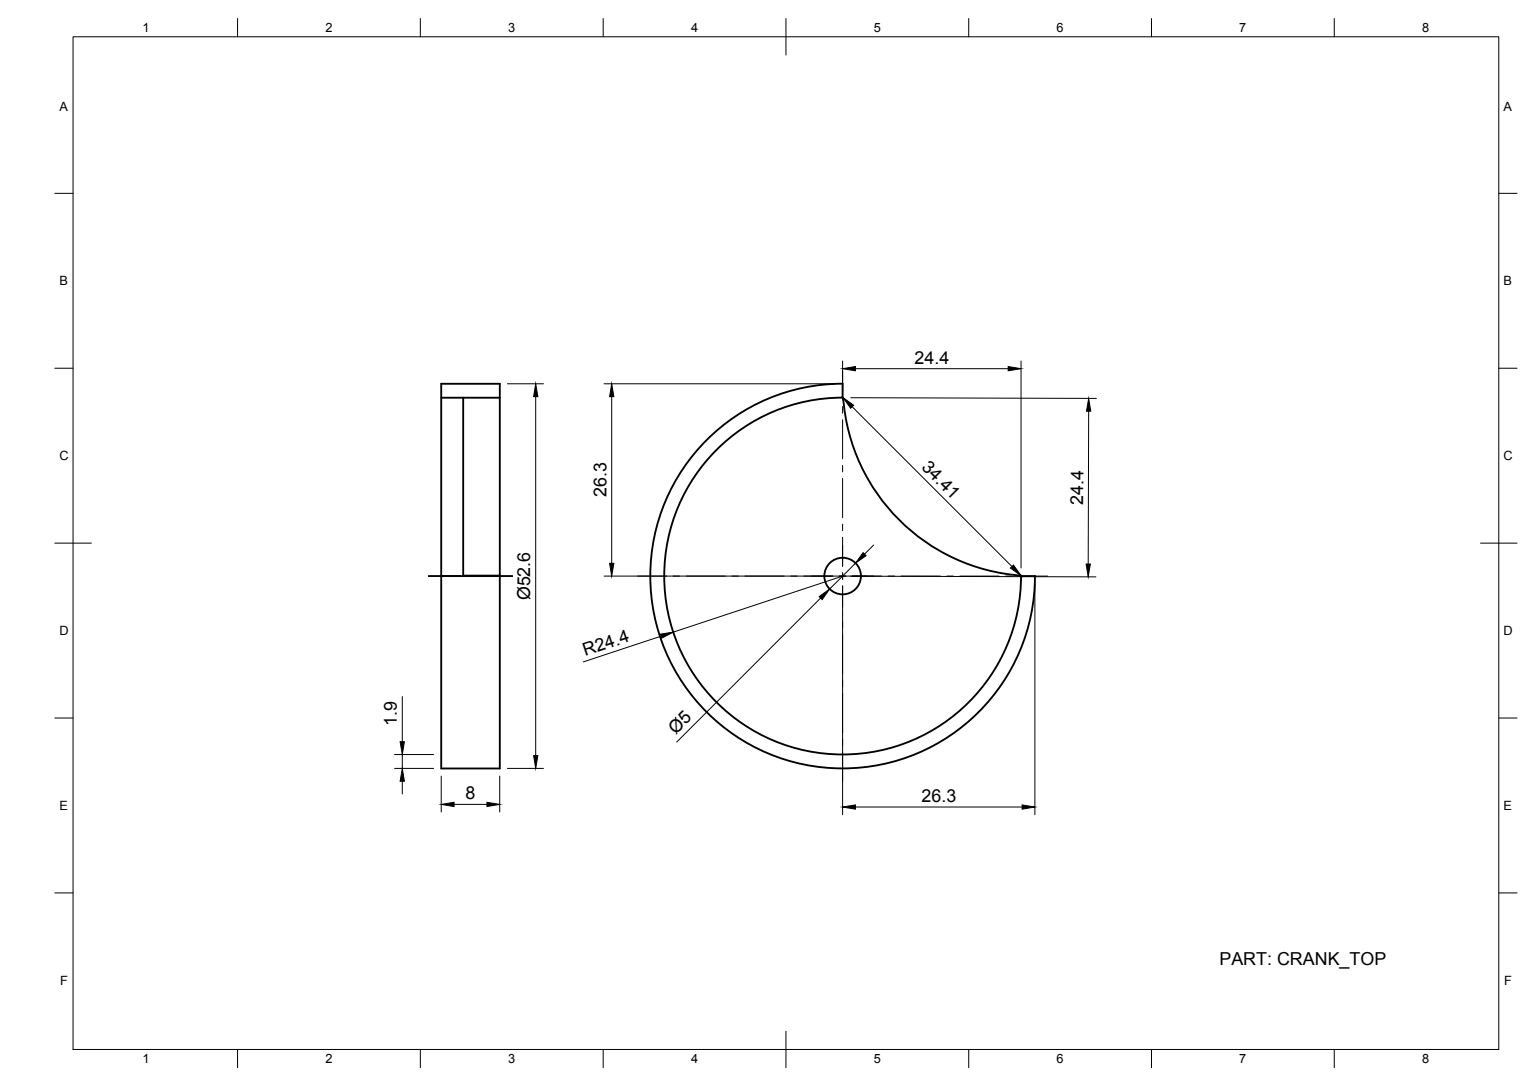
ISO-10303-21;
HEADER;
/* Generated by software containing ST-Developer
 * from STEP Tools, Inc. (www.steptools.com) 
 */

FILE_DESCRIPTION(
/* description */ (''),
/* implementation_level */ '2;1');

FILE_NAME(
/* name */ 'Crank_Top.step',
/* time_stamp */ '2026-09-20T21:52:48+06:00',
/* author */ (''),
/* organization */ (''),
/* preprocessor_version */ 'ST-DEVELOPER v20.2',
/* originating_system */ 'Autodesk Translation Framework v15.15.0.0',
/* authorisation */ '');

FILE_SCHEMA (('AUTOMOTIVE_DESIGN { 1 0 10303 214 3 1 1 }'));
ENDSEC;

DATA;
#10=MECHANICAL_DESIGN_GEOMETRIC_PRESENTATION_REPRESENTATION('',(#64),#2203);
#48=SHAPE_REPRESENTATION_RELATIONSHIP('SRR','None',#2240,#56);
#56=ADVANCED_BREP_SHAPE_REPRESENTATION('',(#72),#2200);
#64=STYLED_ITEM('',(#2285),#72);
#72=MANIFOLD_SOLID_BREP('Crank_Top',#1231);
#85=FACE_BOUND('',#297,.T.);
#86=FACE_BOUND('',#303,.T.);
#123=CIRCLE('',#1417,24.399223777829);
#124=CIRCLE('',#1418,26.3);
#125=CIRCLE('',#1420,24.399223777829);
#126=CIRCLE('',#1422,26.3);
#127=CIRCLE('',#1425,26.3);
#128=CIRCLE('',#1426,2.5);
#129=CIRCLE('',#1428,26.3);
#130=CIRCLE('',#1430,2.5);
#154=CYLINDRICAL_SURFACE('',#1419,24.399223777829);
#155=CYLINDRICAL_SURFACE('',#1421,26.3);
#156=CYLINDRICAL_SURFACE('',#1427,26.3);
#157=CYLINDRICAL_SURFACE('',#1429,2.5);
#212=FACE_OUTER_BOUND('',#291,.T.);
#213=FACE_OUTER_BOUND('',#292,.T.);
#214=FACE_OUTER_BOUND('',#293,.T.);
#215=FACE_OUTER_BOUND('',#294,.T.);
#216=FACE_OUTER_BOUND('',#295,.T.);
#217=FACE_OUTER_BOUND('',#296,.T.);
#218=FACE_OUTER_BOUND('',#298,.T.);
#219=FACE_OUTER_BOUND('',#299,.T.);
#220=FACE_OUTER_BOUND('',#300,.T.);
#221=FACE_OUTER_BOUND('',#301,.T.);
#222=FACE_OUTER_BOUND('',#302,.T.);
#291=EDGE_LOOP('',(#1042,#1043,#1044,#1045,#1046));
#292=EDGE_LOOP('',(#1047,#1048,#1049,#1050));
#293=EDGE_LOOP('',(#1051,#1052,#1053,#1054));
#294=EDGE_LOOP('',(#1055,#1056,#1057,#1058));
#295=EDGE_LOOP('',(#1059,#1060,#1061,#1062));
#296=EDGE_LOOP('',(#1063,#1064,#1065,#1066,#1067,#1068));
#297=EDGE_LOOP('',(#1069));
#298=EDGE_LOOP('',(#1070,#1071,#1072,#1073));
#299=EDGE_LOOP('',(#1074,#1075,#1076,#1077));
#300=EDGE_LOOP('',(#1078,#1079,#1080,#1081,#1082,#1083));
#301=EDGE_LOOP('',(#1084,#1085,#1086,#1087));
#302=EDGE_LOOP('',(#1088,#1089,#1090,#1091,#1092));
#303=EDGE_LOOP('',(#1093));
#402=LINE('',#2101,#512);
#403=LINE('',#2103,#513);
#404=LINE('',#2105,#514);
#405=LINE('',#2107,#515);
#406=LINE('',#2108,#516);
#407=LINE('',#2113,#517);
#408=LINE('',#2118,#518);
#409=LINE('',#2121,#519);
#410=LINE('',#2126,#520);
#411=LINE('',#2128,#521);
#412=LINE('',#2130,#522);
#413=LINE('',#2131,#523);
#414=LINE('',#2134,#524);
#415=LINE('',#2135,#525);
#416=LINE('',#2141,#526);
#417=LINE('',#2146,#527);
#418=LINE('',#2148,#528);
#419=LINE('',#2150,#529);
#512=VECTOR('',#1732,10.);
#513=VECTOR('',#1733,10.);
#514=VECTOR('',#1734,10.);
#515=VECTOR('',#1735,10.);
#516=VECTOR('',#1736,10.);
#517=VECTOR('',#1741,10.);
#518=VECTOR('',#1748,10.);
#519=VECTOR('',#1751,10.);
#520=VECTOR('',#1756,10.);
#521=VECTOR('',#1757,10.);
#522=VECTOR('',#1758,10.);
#523=VECTOR('',#1759,10.);
#524=VECTOR('',#1762,10.);
#525=VECTOR('',#1763,10.);
#526=VECTOR('',#1770,10.);
#527=VECTOR('',#1777,2.5);
#528=VECTOR('',#1780,10.);
#529=VECTOR('',#1783,10.);
#615=VERTEX_POINT('',#2099);
#616=VERTEX_POINT('',#2100);
#617=VERTEX_POINT('',#2102);
#618=VERTEX_POINT('',#2104);
#619=VERTEX_POINT('',#2106);
#620=VERTEX_POINT('',#2110);
#621=VERTEX_POINT('',#2112);
#622=VERTEX_POINT('',#2116);
#623=VERTEX_POINT('',#2120);
#624=VERTEX_POINT('',#2124);
#625=VERTEX_POINT('',#2125);
#626=VERTEX_POINT('',#2127);
#627=VERTEX_POINT('',#2129);
#628=VERTEX_POINT('',#2133);
#629=VERTEX_POINT('',#2137);
#630=VERTEX_POINT('',#2140);
#631=VERTEX_POINT('',#2144);
#761=EDGE_CURVE('',#615,#616,#402,.T.);
#762=EDGE_CURVE('',#617,#615,#403,.T.);
#763=EDGE_CURVE('',#618,#617,#404,.T.);
#764=EDGE_CURVE('',#619,#618,#405,.T.);
#765=EDGE_CURVE('',#619,#616,#406,.T.);
#766=EDGE_CURVE('',#615,#620,#123,.T.);
#767=EDGE_CURVE('',#620,#621,#407,.T.);
#768=EDGE_CURVE('',#621,#617,#124,.T.);
#769=EDGE_CURVE('',#622,#616,#125,.T.);
#770=EDGE_CURVE('',#620,#622,#408,.T.);
#771=EDGE_CURVE('',#621,#623,#409,.T.);
#772=EDGE_CURVE('',#618,#623,#126,.T.);
#773=EDGE_CURVE('',#624,#625,#410,.T.);
#774=EDGE_CURVE('',#626,#624,#411,.T.);
#775=EDGE_CURVE('',#627,#626,#412,.T.);
#776=EDGE_CURVE('',#627,#625,#413,.T.);
#777=EDGE_CURVE('',#628,#619,#414,.T.);
#778=EDGE_CURVE('',#623,#627,#415,.T.);
#779=EDGE_CURVE('',#626,#628,#127,.T.);
#780=EDGE_CURVE('',#629,#629,#128,.T.);
#781=EDGE_CURVE('',#630,#628,#416,.T.);
#782=EDGE_CURVE('',#624,#630,#129,.T.);
#783=EDGE_CURVE('',#631,#631,#130,.T.);
#784=EDGE_CURVE('',#631,#629,#417,.T.);
#785=EDGE_CURVE('',#625,#622,#418,.T.);
#786=EDGE_CURVE('',#616,#630,#419,.T.);
#1042=ORIENTED_EDGE('',*,*,#761,.F.);
#1043=ORIENTED_EDGE('',*,*,#762,.F.);
#1044=ORIENTED_EDGE('',*,*,#763,.F.);
#1045=ORIENTED_EDGE('',*,*,#764,.F.);
#1046=ORIENTED_EDGE('',*,*,#765,.T.);
#1047=ORIENTED_EDGE('',*,*,#762,.T.);
#1048=ORIENTED_EDGE('',*,*,#766,.T.);
#1049=ORIENTED_EDGE('',*,*,#767,.T.);
#1050=ORIENTED_EDGE('',*,*,#768,.T.);
#1051=ORIENTED_EDGE('',*,*,#769,.F.);
#1052=ORIENTED_EDGE('',*,*,#770,.F.);
#1053=ORIENTED_EDGE('',*,*,#766,.F.);
#1054=ORIENTED_EDGE('',*,*,#761,.T.);
#1055=ORIENTED_EDGE('',*,*,#763,.T.);
#1056=ORIENTED_EDGE('',*,*,#768,.F.);
#1057=ORIENTED_EDGE('',*,*,#771,.T.);
#1058=ORIENTED_EDGE('',*,*,#772,.F.);
#1059=ORIENTED_EDGE('',*,*,#773,.F.);
#1060=ORIENTED_EDGE('',*,*,#774,.F.);
#1061=ORIENTED_EDGE('',*,*,#775,.F.);
#1062=ORIENTED_EDGE('',*,*,#776,.T.);
#1063=ORIENTED_EDGE('',*,*,#777,.T.);
#1064=ORIENTED_EDGE('',*,*,#764,.T.);
#1065=ORIENTED_EDGE('',*,*,#772,.T.);
#1066=ORIENTED_EDGE('',*,*,#778,.T.);
#1067=ORIENTED_EDGE('',*,*,#775,.T.);
#1068=ORIENTED_EDGE('',*,*,#779,.T.);
#1069=ORIENTED_EDGE('',*,*,#780,.T.);
#1070=ORIENTED_EDGE('',*,*,#781,.T.);
#1071=ORIENTED_EDGE('',*,*,#779,.F.);
#1072=ORIENTED_EDGE('',*,*,#774,.T.);
#1073=ORIENTED_EDGE('',*,*,#782,.T.);
#1074=ORIENTED_EDGE('',*,*,#783,.F.);
#1075=ORIENTED_EDGE('',*,*,#784,.T.);
#1076=ORIENTED_EDGE('',*,*,#780,.F.);
#1077=ORIENTED_EDGE('',*,*,#784,.F.);
#1078=ORIENTED_EDGE('',*,*,#785,.F.);
#1079=ORIENTED_EDGE('',*,*,#776,.F.);
#1080=ORIENTED_EDGE('',*,*,#778,.F.);
#1081=ORIENTED_EDGE('',*,*,#771,.F.);
#1082=ORIENTED_EDGE('',*,*,#767,.F.);
#1083=ORIENTED_EDGE('',*,*,#770,.T.);
#1084=ORIENTED_EDGE('',*,*,#786,.F.);
#1085=ORIENTED_EDGE('',*,*,#765,.F.);
#1086=ORIENTED_EDGE('',*,*,#777,.F.);
#1087=ORIENTED_EDGE('',*,*,#781,.F.);
#1088=ORIENTED_EDGE('',*,*,#785,.T.);
#1089=ORIENTED_EDGE('',*,*,#769,.T.);
#1090=ORIENTED_EDGE('',*,*,#786,.T.);
#1091=ORIENTED_EDGE('',*,*,#782,.F.);
#1092=ORIENTED_EDGE('',*,*,#773,.T.);
#1093=ORIENTED_EDGE('',*,*,#783,.T.);
#1146=PLANE('',#1415);
#1147=PLANE('',#1416);
#1148=PLANE('',#1423);
#1149=PLANE('',#1424);
#1150=PLANE('',#1431);
#1151=PLANE('',#1432);
#1152=PLANE('',#1433);
#1208=ADVANCED_FACE('',(#212),#1146,.F.);
#1209=ADVANCED_FACE('',(#213),#1147,.T.);
#1210=ADVANCED_FACE('',(#214),#154,.F.);
#1211=ADVANCED_FACE('',(#215),#155,.T.);
#1212=ADVANCED_FACE('',(#216),#1148,.T.);
#1213=ADVANCED_FACE('',(#217,#85),#1149,.F.);
#1214=ADVANCED_FACE('',(#218),#156,.F.);
#1215=ADVANCED_FACE('',(#219),#157,.F.);
#1216=ADVANCED_FACE('',(#220),#1150,.T.);
#1217=ADVANCED_FACE('',(#221),#1151,.F.);
#1218=ADVANCED_FACE('',(#222,#86),#1152,.T.);
#1231=CLOSED_SHELL('',(#1208,#1209,#1210,#1211,#1212,#1213,#1214,#1215,
#1216,#1217,#1218));
#1414=AXIS2_PLACEMENT_3D('',#2097,#1728,#1729);
#1415=AXIS2_PLACEMENT_3D('',#2098,#1730,#1731);
#1416=AXIS2_PLACEMENT_3D('',#2109,#1737,#1738);
#1417=AXIS2_PLACEMENT_3D('',#2111,#1739,#1740);
#1418=AXIS2_PLACEMENT_3D('',#2114,#1742,#1743);
#1419=AXIS2_PLACEMENT_3D('',#2115,#1744,#1745);
#1420=AXIS2_PLACEMENT_3D('',#2117,#1746,#1747);
#1421=AXIS2_PLACEMENT_3D('',#2119,#1749,#1750);
#1422=AXIS2_PLACEMENT_3D('',#2122,#1752,#1753);
#1423=AXIS2_PLACEMENT_3D('',#2123,#1754,#1755);
#1424=AXIS2_PLACEMENT_3D('',#2132,#1760,#1761);
#1425=AXIS2_PLACEMENT_3D('',#2136,#1764,#1765);
#1426=AXIS2_PLACEMENT_3D('',#2138,#1766,#1767);
#1427=AXIS2_PLACEMENT_3D('',#2139,#1768,#1769);
#1428=AXIS2_PLACEMENT_3D('',#2142,#1771,#1772);
#1429=AXIS2_PLACEMENT_3D('',#2143,#1773,#1774);
#1430=AXIS2_PLACEMENT_3D('',#2145,#1775,#1776);
#1431=AXIS2_PLACEMENT_3D('',#2147,#1778,#1779);
#1432=AXIS2_PLACEMENT_3D('',#2149,#1781,#1782);
#1433=AXIS2_PLACEMENT_3D('',#2151,#1784,#1785);
#1728=DIRECTION('axis',(0.,0.,1.));
#1729=DIRECTION('refdir',(1.,0.,0.));
#1730=DIRECTION('center_axis',(-1.,0.,0.));
#1731=DIRECTION('ref_axis',(0.,0.,1.));
#1732=DIRECTION('',(0.,-1.,0.));
#1733=DIRECTION('',(0.,0.,-1.));
#1734=DIRECTION('',(0.,1.,0.));
#1735=DIRECTION('',(0.,0.,1.));
#1736=DIRECTION('',(0.,1.,0.));
#1737=DIRECTION('center_axis',(0.,1.,0.));
#1738=DIRECTION('ref_axis',(1.,0.,0.));
#1739=DIRECTION('center_axis',(0.,-1.,0.));
#1740=DIRECTION('ref_axis',(-1.,0.,0.));
#1741=DIRECTION('',(1.,0.,0.));
#1742=DIRECTION('center_axis',(0.,1.,0.));
#1743=DIRECTION('ref_axis',(1.,0.,0.));
#1744=DIRECTION('center_axis',(0.,1.,0.));
#1745=DIRECTION('ref_axis',(-1.,0.,0.));
#1746=DIRECTION('center_axis',(0.,1.,0.));
#1747=DIRECTION('ref_axis',(-1.,0.,0.));
#1748=DIRECTION('',(0.,-1.,0.));
#1749=DIRECTION('center_axis',(0.,1.,0.));
#1750=DIRECTION('ref_axis',(-0.707106781186548,0.,-0.707106781186547));
#1751=DIRECTION('',(0.,-1.,0.));
#1752=DIRECTION('center_axis',(0.,-1.,0.));
#1753=DIRECTION('ref_axis',(1.,0.,0.));
#1754=DIRECTION('center_axis',(0.983844577872192,0.,-0.179024709443944));
#1755=DIRECTION('ref_axis',(-0.179024709443944,0.,-0.983844577872192));
#1756=DIRECTION('',(-0.179024709443944,0.,-0.983844577872192));
#1757=DIRECTION('',(0.,1.,0.));
#1758=DIRECTION('',(0.179024709443944,0.,0.983844577872192));
#1759=DIRECTION('',(0.,1.,0.));
#1760=DIRECTION('center_axis',(0.,1.,0.));
#1761=DIRECTION('ref_axis',(1.,0.,0.));
#1762=DIRECTION('',(-0.999999006571221,0.,0.00140955899906737));
#1763=DIRECTION('',(-1.,0.,0.));
#1764=DIRECTION('center_axis',(0.,1.,0.));
#1765=DIRECTION('ref_axis',(3.37710425741493E-16,0.,-1.));
#1766=DIRECTION('center_axis',(0.,1.,0.));
#1767=DIRECTION('ref_axis',(1.,0.,0.));
#1768=DIRECTION('center_axis',(0.,1.,0.));
#1769=DIRECTION('ref_axis',(3.37710425741493E-16,0.,-1.));
#1770=DIRECTION('',(0.,-1.,0.));
#1771=DIRECTION('center_axis',(0.,1.,0.));
#1772=DIRECTION('ref_axis',(3.37710425741493E-16,0.,-1.));
#1773=DIRECTION('center_axis',(0.,1.,0.));
#1774=DIRECTION('ref_axis',(1.,0.,0.));
#1775=DIRECTION('center_axis',(0.,-1.,0.));
#1776=DIRECTION('ref_axis',(1.,0.,0.));
#1777=DIRECTION('',(0.,-1.,0.));
#1778=DIRECTION('center_axis',(0.,0.,1.));
#1779=DIRECTION('ref_axis',(1.,0.,0.));
#1780=DIRECTION('',(1.,0.,0.));
#1781=DIRECTION('center_axis',(-0.00140955899906737,0.,-0.999999006571221));
#1782=DIRECTION('ref_axis',(-0.999999006571221,0.,0.00140955899906737));
#1783=DIRECTION('',(0.999999006571221,0.,-0.00140955899906737));
#1784=DIRECTION('center_axis',(0.,1.,0.));
#1785=DIRECTION('ref_axis',(0.,0.,1.));
#2097=CARTESIAN_POINT('',(0.,0.,0.));
#2098=CARTESIAN_POINT('Origin',(0.,3.,26.3));
#2099=CARTESIAN_POINT('',(0.,3.,50.699223777829));
#2100=CARTESIAN_POINT('',(0.,0.,50.699223777829));
#2101=CARTESIAN_POINT('',(0.,3.,50.699223777829));
#2102=CARTESIAN_POINT('',(4.16333634234434E-15,3.,52.6));
#2103=CARTESIAN_POINT('',(0.,3.,33.4516927808502));
#2104=CARTESIAN_POINT('',(4.16333634234434E-15,-5.,52.6));
#2105=CARTESIAN_POINT('',(4.44089209850063E-15,0.,52.6));
#2106=CARTESIAN_POINT('',(0.,-5.,50.699223777829));
#2107=CARTESIAN_POINT('',(0.,-5.,26.3));
#2108=CARTESIAN_POINT('',(0.,3.,50.699223777829));
#2109=CARTESIAN_POINT('Origin',(14.3033855617004,3.,40.6033855617004));
#2110=CARTESIAN_POINT('',(24.399223777829,3.,26.3));
#2111=CARTESIAN_POINT('Origin',(0.,3.,26.3));
#2112=CARTESIAN_POINT('',(26.3,3.,26.3));
#2113=CARTESIAN_POINT('',(0.,3.,26.3));
#2114=CARTESIAN_POINT('Origin',(0.,3.,26.3));
#2115=CARTESIAN_POINT('Origin',(0.,3.,26.3));
#2116=CARTESIAN_POINT('',(24.399223777829,0.,26.3));
#2117=CARTESIAN_POINT('Origin',(0.,0.,26.3));
#2118=CARTESIAN_POINT('',(24.399223777829,3.,26.3));
#2119=CARTESIAN_POINT('Origin',(0.,0.,26.3));
#2120=CARTESIAN_POINT('',(26.3,-5.,26.3));
#2121=CARTESIAN_POINT('',(26.3,0.,26.3));
#2122=CARTESIAN_POINT('Origin',(0.,-5.,26.3));
#2123=CARTESIAN_POINT('Origin',(27.8026817657391,0.,45.0732920359323));
#2124=CARTESIAN_POINT('',(24.3991268223128,0.,26.3687842225651));
#2125=CARTESIAN_POINT('',(24.3866105410464,0.,26.3));
#2126=CARTESIAN_POINT('',(25.9192569340967,0.,34.7227805663332));
#2127=CARTESIAN_POINT('',(24.3991268223128,-5.,26.3687842225651));
#2128=CARTESIAN_POINT('',(24.3991268223128,0.,26.3687842225651));
#2129=CARTESIAN_POINT('',(24.3866105410464,-5.,26.3));
#2130=CARTESIAN_POINT('',(24.3866105410464,-5.,26.3));
#2131=CARTESIAN_POINT('',(24.3866105410464,0.,26.3));
#2132=CARTESIAN_POINT('Origin',(0.,-5.,26.3));
#2133=CARTESIAN_POINT('',(0.0687842225651092,-5.,50.6991268223128));
#2134=CARTESIAN_POINT('',(0.0515881669226298,-5.,50.6991510611919));
#2135=CARTESIAN_POINT('',(0.,-5.,26.3));
#2136=CARTESIAN_POINT('Origin',(26.3,-5.,52.6));
#2137=CARTESIAN_POINT('',(-2.5,-5.,26.3));
#2138=CARTESIAN_POINT('Origin',(0.,-5.,26.3));
#2139=CARTESIAN_POINT('Origin',(26.3,0.,52.6));
#2140=CARTESIAN_POINT('',(0.0687842225651092,0.,50.6991268223128));
#2141=CARTESIAN_POINT('',(0.0687842225651059,0.,50.6991268223128));
#2142=CARTESIAN_POINT('Origin',(26.3,0.,52.6));
#2143=CARTESIAN_POINT('Origin',(0.,0.,26.3));
#2144=CARTESIAN_POINT('',(-2.5,0.,26.3));
#2145=CARTESIAN_POINT('Origin',(0.,0.,26.3));
#2146=CARTESIAN_POINT('',(-2.5,0.,26.3));
#2147=CARTESIAN_POINT('Origin',(24.3866105410464,0.,26.3));
#2148=CARTESIAN_POINT('',(13.2279960512749,0.,26.3));
#2149=CARTESIAN_POINT('Origin',(0.0687842225651092,-5.,50.6991268223128));
#2150=CARTESIAN_POINT('',(1.08481843563973,0.,50.6976946607217));
#2151=CARTESIAN_POINT('Origin',(2.06938156150334,0.,28.3693815615033));
#2190=UNCERTAINTY_MEASURE_WITH_UNIT(LENGTH_MEASURE(0.01),#2204,
'DISTANCE_ACCURACY_VALUE',
'Maximum model space distance between geometric entities at asserted c
onnectivities');
#2193=UNCERTAINTY_MEASURE_WITH_UNIT(LENGTH_MEASURE(0.01),#2204,
'DISTANCE_ACCURACY_VALUE',
'Maximum model space distance between geometric entities at asserted c
onnectivities');
#2200=(
GEOMETRIC_REPRESENTATION_CONTEXT(3)
GLOBAL_UNCERTAINTY_ASSIGNED_CONTEXT((#2190))
GLOBAL_UNIT_ASSIGNED_CONTEXT((#2204,#2206,#2207))
REPRESENTATION_CONTEXT('','3D')
);
#2203=(
GEOMETRIC_REPRESENTATION_CONTEXT(3)
GLOBAL_UNCERTAINTY_ASSIGNED_CONTEXT((#2193))
GLOBAL_UNIT_ASSIGNED_CONTEXT((#2204,#2206,#2207))
REPRESENTATION_CONTEXT('','3D')
);
#2204=(
LENGTH_UNIT()
NAMED_UNIT(*)
SI_UNIT(.MILLI.,.METRE.)
);
#2206=(
NAMED_UNIT(*)
PLANE_ANGLE_UNIT()
SI_UNIT($,.RADIAN.)
);
#2207=(
NAMED_UNIT(*)
SI_UNIT($,.STERADIAN.)
SOLID_ANGLE_UNIT()
);
#2214=SHAPE_DEFINITION_REPRESENTATION(#2223,#2240);
#2223=PRODUCT_DEFINITION_SHAPE('',$,#2250);
#2240=SHAPE_REPRESENTATION('',(#1414),#2200);
#2243=PRODUCT_DEFINITION_CONTEXT('part definition',#2272,'design');
#2250=PRODUCT_DEFINITION('Crank_Top','Crank_Top',#2259,#2243);
#2259=PRODUCT_DEFINITION_FORMATION('',$,#2280);
#2272=APPLICATION_CONTEXT(
'Core Data for Automotive Mechanical Design Process');
#2273=PRODUCT_CONTEXT('part definition',#2272,'mechanical');
#2280=PRODUCT('Crank_Top','Crank_Top',$,(#2273));
#2285=PRESENTATION_STYLE_ASSIGNMENT((#2289));
#2289=SURFACE_STYLE_USAGE(.BOTH.,#2293);
#2293=SURFACE_SIDE_STYLE('',(#2297));
#2297=SURFACE_STYLE_FILL_AREA(#2301);
#2301=FILL_AREA_STYLE('Surface - Matte',(#2305));
#2305=FILL_AREA_STYLE_COLOUR('Surface - Matte',#2309);
#2309=COLOUR_RGB('Surface - Matte', 0.66274510, 0.83137255, 0.94901961);
ENDSEC;
END-ISO-10303-21;
